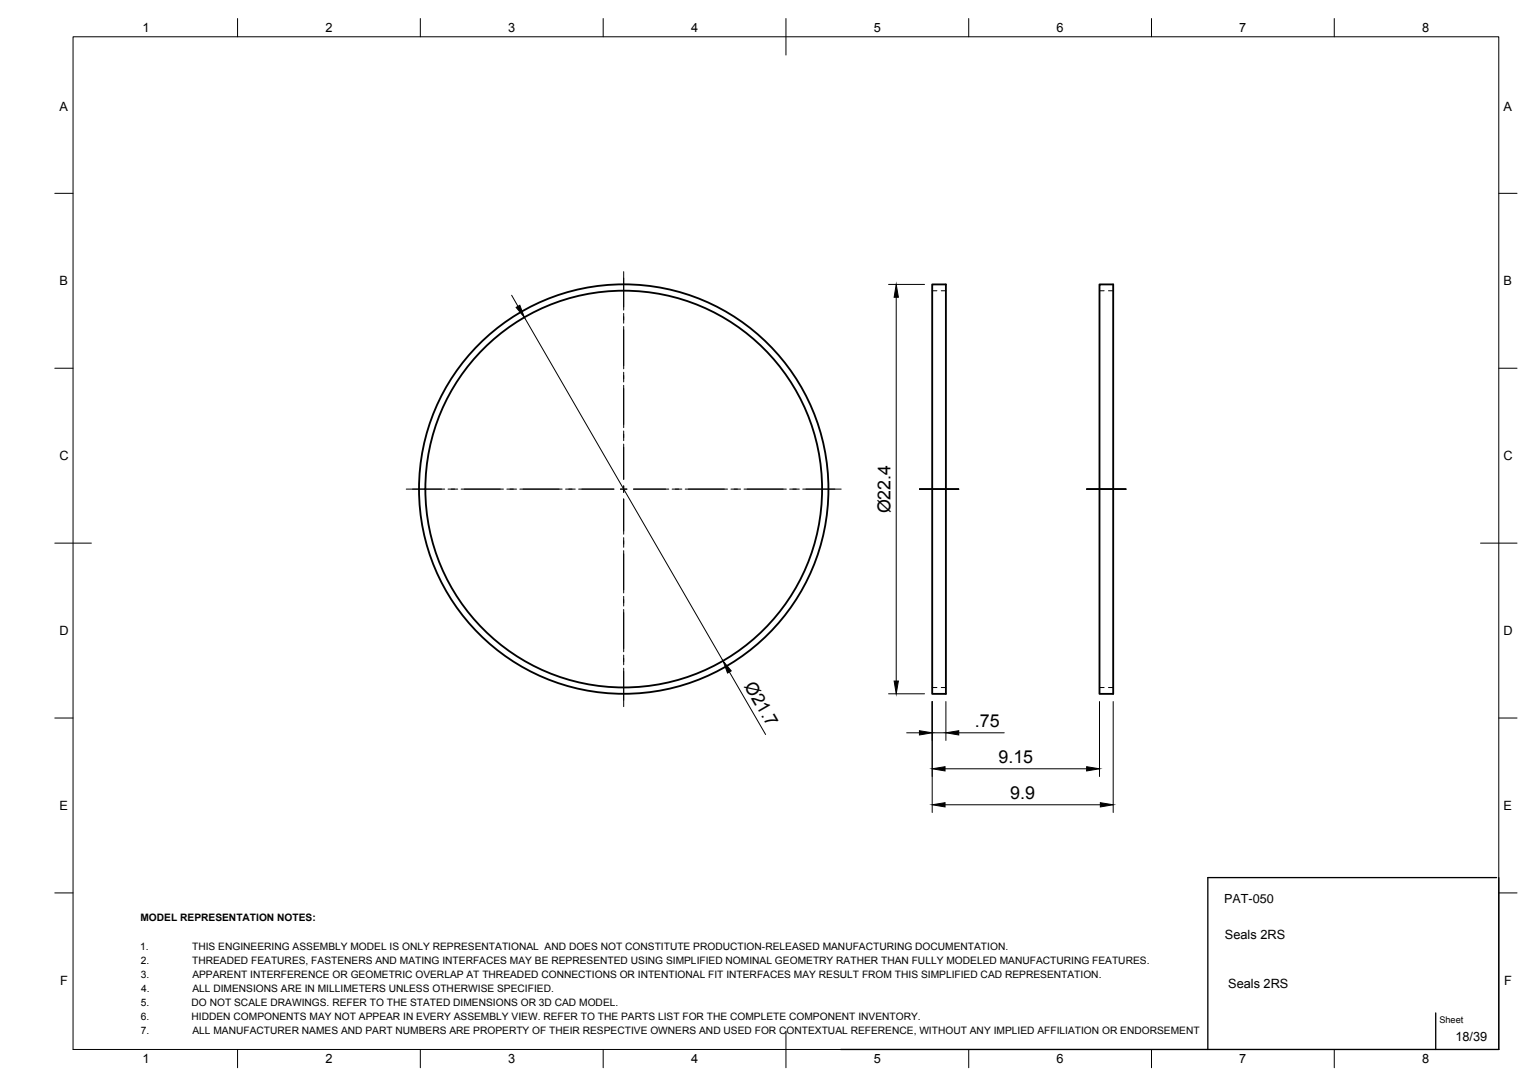
ISO-10303-21;
HEADER;
/* Generated by software containing ST-Developer
 * from STEP Tools, Inc. (www.steptools.com) 
 */

FILE_DESCRIPTION(
/* description */ ('Hand wheel with handle and shaft collar'),
/* implementation_level */ '2;1');

FILE_NAME(
/* name */ 'Seals 2RS.step',
/* time_stamp */ '2026-10-28T03:23:19-07:00',
/* author */ (''),
/* organization */ (''),
/* preprocessor_version */ 'ST-DEVELOPER v20.2',
/* originating_system */ 'Autodesk Translation Framework v15.17.0.0',
/* authorisation */ '');

FILE_SCHEMA (('AUTOMOTIVE_DESIGN { 1 0 10303 214 3 1 1 }'));
ENDSEC;

DATA;
#10=MECHANICAL_DESIGN_GEOMETRIC_PRESENTATION_REPRESENTATION('',(#414,#415),#10510);
#344=SHAPE_REPRESENTATION_RELATIONSHIP('SRR','None',#10661,#376);
#376=ADVANCED_BREP_SHAPE_REPRESENTATION('',(#460,#461),#10488);
#414=STYLED_ITEM('',(#10908),#460);
#415=STYLED_ITEM('',(#10908),#461);
#460=MANIFOLD_SOLID_BREP('Body1',#5314);
#461=MANIFOLD_SOLID_BREP('Body2',#5315);
#544=FACE_BOUND('',#1266,.T.);
#545=FACE_BOUND('',#1269,.T.);
#546=FACE_BOUND('',#1272,.T.);
#547=FACE_BOUND('',#1275,.T.);
#659=PLANE('',#5969);
#660=PLANE('',#5974);
#661=PLANE('',#5977);
#662=PLANE('',#5982);
#888=FACE_OUTER_BOUND('',#1265,.T.);
#889=FACE_OUTER_BOUND('',#1267,.T.);
#890=FACE_OUTER_BOUND('',#1268,.T.);
#891=FACE_OUTER_BOUND('',#1270,.T.);
#892=FACE_OUTER_BOUND('',#1271,.T.);
#893=FACE_OUTER_BOUND('',#1273,.T.);
#894=FACE_OUTER_BOUND('',#1274,.T.);
#895=FACE_OUTER_BOUND('',#1276,.T.);
#1265=EDGE_LOOP('',(#4097));
#1266=EDGE_LOOP('',(#4098));
#1267=EDGE_LOOP('',(#4099,#4100,#4101,#4102));
#1268=EDGE_LOOP('',(#4103));
#1269=EDGE_LOOP('',(#4104));
#1270=EDGE_LOOP('',(#4105,#4106,#4107,#4108));
#1271=EDGE_LOOP('',(#4109));
#1272=EDGE_LOOP('',(#4110));
#1273=EDGE_LOOP('',(#4111,#4112,#4113,#4114));
#1274=EDGE_LOOP('',(#4115));
#1275=EDGE_LOOP('',(#4116));
#1276=EDGE_LOOP('',(#4117,#4118,#4119,#4120));
#1639=LINE('',#9074,#1949);
#1640=LINE('',#9079,#1950);
#1641=LINE('',#9088,#1951);
#1642=LINE('',#9093,#1952);
#1949=VECTOR('',#7099,1.119765);
#1950=VECTOR('',#7106,1.085235);
#1951=VECTOR('',#7117,1.119765);
#1952=VECTOR('',#7124,1.085235);
#2263=CIRCLE('',#5970,1.119765);
#2264=CIRCLE('',#5971,1.085235);
#2265=CIRCLE('',#5973,1.119765);
#2266=CIRCLE('',#5975,1.085235);
#2267=CIRCLE('',#5978,1.119765);
#2268=CIRCLE('',#5979,1.085235);
#2269=CIRCLE('',#5981,1.119765);
#2270=CIRCLE('',#5983,1.085235);
#2631=VERTEX_POINT('',#9067);
#2632=VERTEX_POINT('',#9069);
#2633=VERTEX_POINT('',#9072);
#2634=VERTEX_POINT('',#9076);
#2635=VERTEX_POINT('',#9081);
#2636=VERTEX_POINT('',#9083);
#2637=VERTEX_POINT('',#9086);
#2638=VERTEX_POINT('',#9090);
#3166=EDGE_CURVE('',#2631,#2631,#2263,.T.);
#3167=EDGE_CURVE('',#2632,#2632,#2264,.T.);
#3168=EDGE_CURVE('',#2633,#2633,#2265,.T.);
#3169=EDGE_CURVE('',#2633,#2631,#1639,.T.);
#3170=EDGE_CURVE('',#2634,#2634,#2266,.T.);
#3171=EDGE_CURVE('',#2634,#2632,#1640,.T.);
#3172=EDGE_CURVE('',#2635,#2635,#2267,.T.);
#3173=EDGE_CURVE('',#2636,#2636,#2268,.T.);
#3174=EDGE_CURVE('',#2637,#2637,#2269,.T.);
#3175=EDGE_CURVE('',#2637,#2635,#1641,.T.);
#3176=EDGE_CURVE('',#2638,#2638,#2270,.T.);
#3177=EDGE_CURVE('',#2638,#2636,#1642,.T.);
#4097=ORIENTED_EDGE('',*,*,#3166,.F.);
#4098=ORIENTED_EDGE('',*,*,#3167,.T.);
#4099=ORIENTED_EDGE('',*,*,#3168,.F.);
#4100=ORIENTED_EDGE('',*,*,#3169,.T.);
#4101=ORIENTED_EDGE('',*,*,#3166,.T.);
#4102=ORIENTED_EDGE('',*,*,#3169,.F.);
#4103=ORIENTED_EDGE('',*,*,#3168,.T.);
#4104=ORIENTED_EDGE('',*,*,#3170,.F.);
#4105=ORIENTED_EDGE('',*,*,#3170,.T.);
#4106=ORIENTED_EDGE('',*,*,#3171,.T.);
#4107=ORIENTED_EDGE('',*,*,#3167,.F.);
#4108=ORIENTED_EDGE('',*,*,#3171,.F.);
#4109=ORIENTED_EDGE('',*,*,#3172,.F.);
#4110=ORIENTED_EDGE('',*,*,#3173,.T.);
#4111=ORIENTED_EDGE('',*,*,#3174,.F.);
#4112=ORIENTED_EDGE('',*,*,#3175,.T.);
#4113=ORIENTED_EDGE('',*,*,#3172,.T.);
#4114=ORIENTED_EDGE('',*,*,#3175,.F.);
#4115=ORIENTED_EDGE('',*,*,#3174,.T.);
#4116=ORIENTED_EDGE('',*,*,#3176,.F.);
#4117=ORIENTED_EDGE('',*,*,#3176,.T.);
#4118=ORIENTED_EDGE('',*,*,#3177,.T.);
#4119=ORIENTED_EDGE('',*,*,#3173,.F.);
#4120=ORIENTED_EDGE('',*,*,#3177,.F.);
#4920=CYLINDRICAL_SURFACE('',#5972,1.119765);
#4921=CYLINDRICAL_SURFACE('',#5976,1.085235);
#4922=CYLINDRICAL_SURFACE('',#5980,1.119765);
#4923=CYLINDRICAL_SURFACE('',#5984,1.085235);
#5100=ADVANCED_FACE('',(#888,#544),#659,.T.);
#5101=ADVANCED_FACE('',(#889),#4920,.T.);
#5102=ADVANCED_FACE('',(#890,#545),#660,.T.);
#5103=ADVANCED_FACE('',(#891),#4921,.F.);
#5104=ADVANCED_FACE('',(#892,#546),#661,.T.);
#5105=ADVANCED_FACE('',(#893),#4922,.T.);
#5106=ADVANCED_FACE('',(#894,#547),#662,.T.);
#5107=ADVANCED_FACE('',(#895),#4923,.F.);
#5314=CLOSED_SHELL('',(#5100,#5101,#5102,#5103));
#5315=CLOSED_SHELL('',(#5104,#5105,#5106,#5107));
#5968=AXIS2_PLACEMENT_3D('',#9065,#7087,#7088);
#5969=AXIS2_PLACEMENT_3D('',#9066,#7089,#7090);
#5970=AXIS2_PLACEMENT_3D('',#9068,#7091,#7092);
#5971=AXIS2_PLACEMENT_3D('',#9070,#7093,#7094);
#5972=AXIS2_PLACEMENT_3D('',#9071,#7095,#7096);
#5973=AXIS2_PLACEMENT_3D('',#9073,#7097,#7098);
#5974=AXIS2_PLACEMENT_3D('',#9075,#7100,#7101);
#5975=AXIS2_PLACEMENT_3D('',#9077,#7102,#7103);
#5976=AXIS2_PLACEMENT_3D('',#9078,#7104,#7105);
#5977=AXIS2_PLACEMENT_3D('',#9080,#7107,#7108);
#5978=AXIS2_PLACEMENT_3D('',#9082,#7109,#7110);
#5979=AXIS2_PLACEMENT_3D('',#9084,#7111,#7112);
#5980=AXIS2_PLACEMENT_3D('',#9085,#7113,#7114);
#5981=AXIS2_PLACEMENT_3D('',#9087,#7115,#7116);
#5982=AXIS2_PLACEMENT_3D('',#9089,#7118,#7119);
#5983=AXIS2_PLACEMENT_3D('',#9091,#7120,#7121);
#5984=AXIS2_PLACEMENT_3D('',#9092,#7122,#7123);
#7087=DIRECTION('axis',(0.,0.,1.));
#7088=DIRECTION('refdir',(1.,0.,0.));
#7089=DIRECTION('center_axis',(0.,1.,0.));
#7090=DIRECTION('ref_axis',(0.,0.,1.));
#7091=DIRECTION('center_axis',(0.,-1.,0.));
#7092=DIRECTION('ref_axis',(1.,0.,0.));
#7093=DIRECTION('center_axis',(0.,-1.,0.));
#7094=DIRECTION('ref_axis',(1.,0.,0.));
#7095=DIRECTION('center_axis',(0.,-1.,0.));
#7096=DIRECTION('ref_axis',(1.,0.,0.));
#7097=DIRECTION('center_axis',(0.,-1.,0.));
#7098=DIRECTION('ref_axis',(1.,0.,0.));
#7099=DIRECTION('',(0.,1.,0.));
#7100=DIRECTION('center_axis',(0.,-1.,0.));
#7101=DIRECTION('ref_axis',(0.,0.,-1.));
#7102=DIRECTION('center_axis',(0.,-1.,0.));
#7103=DIRECTION('ref_axis',(1.,0.,0.));
#7104=DIRECTION('center_axis',(0.,-1.,0.));
#7105=DIRECTION('ref_axis',(1.,0.,0.));
#7106=DIRECTION('',(0.,1.,0.));
#7107=DIRECTION('center_axis',(0.,1.,0.));
#7108=DIRECTION('ref_axis',(0.,0.,1.));
#7109=DIRECTION('center_axis',(0.,-1.,0.));
#7110=DIRECTION('ref_axis',(1.,0.,0.));
#7111=DIRECTION('center_axis',(0.,-1.,0.));
#7112=DIRECTION('ref_axis',(1.,0.,0.));
#7113=DIRECTION('center_axis',(0.,-1.,0.));
#7114=DIRECTION('ref_axis',(1.,0.,0.));
#7115=DIRECTION('center_axis',(0.,-1.,0.));
#7116=DIRECTION('ref_axis',(1.,0.,0.));
#7117=DIRECTION('',(0.,1.,0.));
#7118=DIRECTION('center_axis',(0.,-1.,0.));
#7119=DIRECTION('ref_axis',(0.,0.,-1.));
#7120=DIRECTION('center_axis',(0.,-1.,0.));
#7121=DIRECTION('ref_axis',(1.,0.,0.));
#7122=DIRECTION('center_axis',(0.,-1.,0.));
#7123=DIRECTION('ref_axis',(1.,0.,0.));
#7124=DIRECTION('',(0.,1.,0.));
#9065=CARTESIAN_POINT('',(0.,0.,0.));
#9066=CARTESIAN_POINT('Origin',(1.119765,0.495,0.));
#9067=CARTESIAN_POINT('',(-1.119765,0.495,-1.37131662304724E-16));
#9068=CARTESIAN_POINT('Origin',(0.,0.495,0.));
#9069=CARTESIAN_POINT('',(-1.085235,0.495,-1.32902956907268E-16));
#9070=CARTESIAN_POINT('Origin',(0.,0.495,0.));
#9071=CARTESIAN_POINT('Origin',(0.,0.4575,0.));
#9072=CARTESIAN_POINT('',(-1.119765,0.42,-1.37131662304724E-16));
#9073=CARTESIAN_POINT('Origin',(0.,0.42,0.));
#9074=CARTESIAN_POINT('',(-1.119765,0.4575,-1.37131662304724E-16));
#9075=CARTESIAN_POINT('Origin',(1.085235,0.42,0.));
#9076=CARTESIAN_POINT('',(-1.085235,0.42,-1.32902956907268E-16));
#9077=CARTESIAN_POINT('Origin',(0.,0.42,0.));
#9078=CARTESIAN_POINT('Origin',(0.,0.4575,0.));
#9079=CARTESIAN_POINT('',(-1.085235,0.4575,-1.32902956907268E-16));
#9080=CARTESIAN_POINT('Origin',(1.119765,-0.42,0.));
#9081=CARTESIAN_POINT('',(-1.119765,-0.42,-1.37131662304724E-16));
#9082=CARTESIAN_POINT('Origin',(0.,-0.42,0.));
#9083=CARTESIAN_POINT('',(-1.085235,-0.42,-1.32902956907268E-16));
#9084=CARTESIAN_POINT('Origin',(0.,-0.42,0.));
#9085=CARTESIAN_POINT('Origin',(0.,-0.4575,0.));
#9086=CARTESIAN_POINT('',(-1.119765,-0.495,-1.37131662304724E-16));
#9087=CARTESIAN_POINT('Origin',(0.,-0.495,0.));
#9088=CARTESIAN_POINT('',(-1.119765,-0.4575,-1.37131662304724E-16));
#9089=CARTESIAN_POINT('Origin',(1.085235,-0.495,0.));
#9090=CARTESIAN_POINT('',(-1.085235,-0.495,-1.32902956907268E-16));
#9091=CARTESIAN_POINT('Origin',(0.,-0.495,0.));
#9092=CARTESIAN_POINT('Origin',(0.,-0.4575,0.));
#9093=CARTESIAN_POINT('',(-1.085235,-0.4575,-1.32902956907268E-16));
#10449=UNCERTAINTY_MEASURE_WITH_UNIT(LENGTH_MEASURE(0.001),#10511,
'DISTANCE_ACCURACY_VALUE',
'Maximum model space distance between geometric entities at asserted c
onnectivities');
#10471=UNCERTAINTY_MEASURE_WITH_UNIT(LENGTH_MEASURE(0.001),#10511,
'DISTANCE_ACCURACY_VALUE',
'Maximum model space distance between geometric entities at asserted c
onnectivities');
#10488=(
GEOMETRIC_REPRESENTATION_CONTEXT(3)
GLOBAL_UNCERTAINTY_ASSIGNED_CONTEXT((#10449))
GLOBAL_UNIT_ASSIGNED_CONTEXT((#10511,#10513,#10514))
REPRESENTATION_CONTEXT('','3D')
);
#10510=(
GEOMETRIC_REPRESENTATION_CONTEXT(3)
GLOBAL_UNCERTAINTY_ASSIGNED_CONTEXT((#10471))
GLOBAL_UNIT_ASSIGNED_CONTEXT((#10511,#10513,#10514))
REPRESENTATION_CONTEXT('','3D')
);
#10511=(
LENGTH_UNIT()
NAMED_UNIT(*)
SI_UNIT(.CENTI.,.METRE.)
);
#10513=(
NAMED_UNIT(*)
PLANE_ANGLE_UNIT()
SI_UNIT($,.RADIAN.)
);
#10514=(
NAMED_UNIT(*)
SI_UNIT($,.STERADIAN.)
SOLID_ANGLE_UNIT()
);
#10531=SHAPE_DEFINITION_REPRESENTATION(#10569,#10661);
#10569=PRODUCT_DEFINITION_SHAPE('',$,#10700);
#10661=SHAPE_REPRESENTATION('',(#5968),#10488);
#10683=PRODUCT_DEFINITION_CONTEXT('part definition',#10799,'design');
#10700=PRODUCT_DEFINITION('Seals 2RS','Seals 2RS',#10738,#10683);
#10738=PRODUCT_DEFINITION_FORMATION('',$,#10817);
#10799=APPLICATION_CONTEXT(
'Core Data for Automotive Mechanical Design Process');
#10800=PRODUCT_CONTEXT('part definition',#10799,'mechanical');
#10817=PRODUCT('Seals 2RS','Seals 2RS','Seals 2RS',(#10800));
#10902=COLOUR_RGB('Grey',0.48,0.52,0.57);
#10903=FILL_AREA_STYLE_COLOUR('',#10902);
#10904=FILL_AREA_STYLE('',(#10903));
#10905=SURFACE_STYLE_FILL_AREA(#10904);
#10906=SURFACE_SIDE_STYLE('',(#10905));
#10907=SURFACE_STYLE_USAGE(.BOTH.,#10906);
#10908=PRESENTATION_STYLE_ASSIGNMENT((#10907));
ENDSEC;
END-ISO-10303-21;
